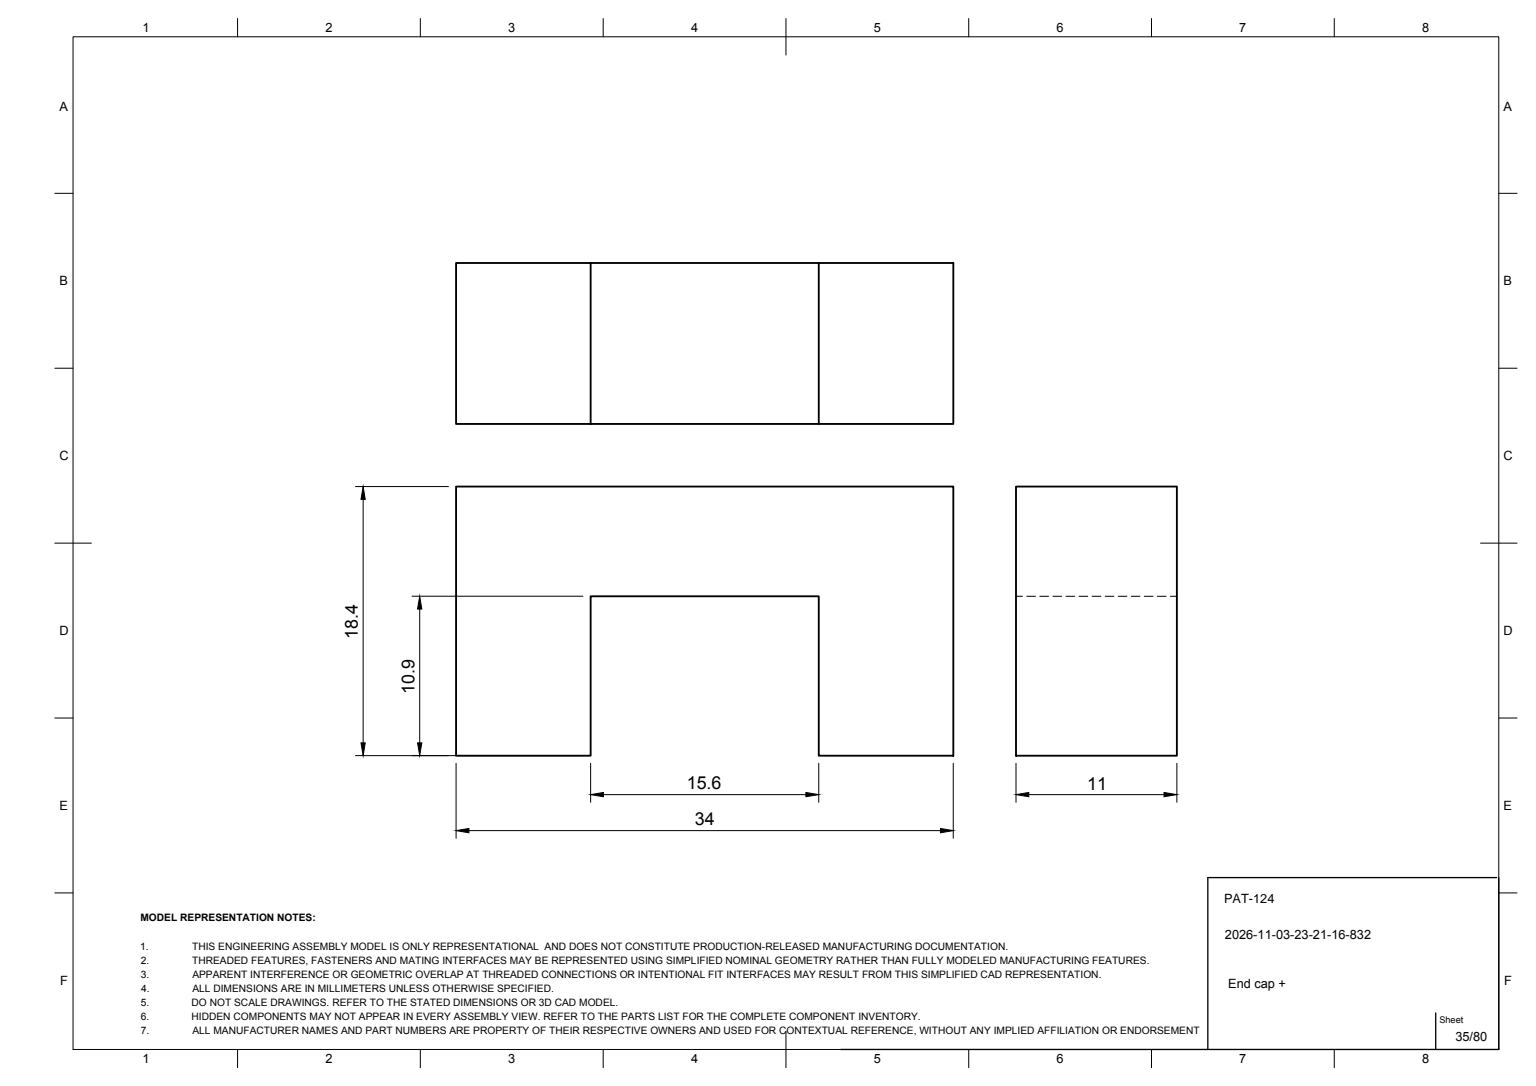
ISO-10303-21;
HEADER;
/* Generated by software containing ST-Developer
 * from STEP Tools, Inc. (www.steptools.com) 
 */

FILE_DESCRIPTION(
/* description */ ('XY cross-slide table'),
/* implementation_level */ '2;1');

FILE_NAME(
/* name */ 'End cap +.step',
/* time_stamp */ '2026-10-28T03:22:46-07:00',
/* author */ (''),
/* organization */ (''),
/* preprocessor_version */ 'ST-DEVELOPER v20.2',
/* originating_system */ 'Autodesk Translation Framework v15.17.0.0',
/* authorisation */ '');

FILE_SCHEMA (('AUTOMOTIVE_DESIGN { 1 0 10303 214 3 1 1 }'));
ENDSEC;

DATA;
#10=MECHANICAL_DESIGN_GEOMETRIC_PRESENTATION_REPRESENTATION('',(#1710),#62984);
#1529=SHAPE_REPRESENTATION_RELATIONSHIP('SRR','None',#63381,#1612);
#1612=ADVANCED_BREP_SHAPE_REPRESENTATION('',(#1823),#62918);
#1710=STYLED_ITEM('',(#63905),#1823);
#1823=MANIFOLD_SOLID_BREP('Body1',#23004);
#2457=PLANE('',#24689);
#2458=PLANE('',#24690);
#2459=PLANE('',#24691);
#2460=PLANE('',#24692);
#2461=PLANE('',#24693);
#2462=PLANE('',#24694);
#2463=PLANE('',#24695);
#2464=PLANE('',#24696);
#2465=PLANE('',#24697);
#2466=PLANE('',#24698);
#3186=FACE_OUTER_BOUND('',#4659,.T.);
#3187=FACE_OUTER_BOUND('',#4660,.T.);
#3188=FACE_OUTER_BOUND('',#4661,.T.);
#3189=FACE_OUTER_BOUND('',#4662,.T.);
#3190=FACE_OUTER_BOUND('',#4663,.T.);
#3191=FACE_OUTER_BOUND('',#4664,.T.);
#3192=FACE_OUTER_BOUND('',#4665,.T.);
#3193=FACE_OUTER_BOUND('',#4666,.T.);
#3194=FACE_OUTER_BOUND('',#4667,.T.);
#3195=FACE_OUTER_BOUND('',#4668,.T.);
#4659=EDGE_LOOP('',(#16324,#16325,#16326,#16327));
#4660=EDGE_LOOP('',(#16328,#16329,#16330,#16331));
#4661=EDGE_LOOP('',(#16332,#16333,#16334,#16335));
#4662=EDGE_LOOP('',(#16336,#16337,#16338,#16339));
#4663=EDGE_LOOP('',(#16340,#16341,#16342,#16343));
#4664=EDGE_LOOP('',(#16344,#16345,#16346,#16347));
#4665=EDGE_LOOP('',(#16348,#16349,#16350,#16351));
#4666=EDGE_LOOP('',(#16352,#16353,#16354,#16355));
#4667=EDGE_LOOP('',(#16356,#16357,#16358,#16359,#16360,#16361,#16362,#16363));
#4668=EDGE_LOOP('',(#16364,#16365,#16366,#16367,#16368,#16369,#16370,#16371));
#6255=LINE('',#35063,#7742);
#6256=LINE('',#35065,#7743);
#6257=LINE('',#35067,#7744);
#6258=LINE('',#35068,#7745);
#6259=LINE('',#35071,#7746);
#6260=LINE('',#35073,#7747);
#6261=LINE('',#35074,#7748);
#6262=LINE('',#35077,#7749);
#6263=LINE('',#35079,#7750);
#6264=LINE('',#35080,#7751);
#6265=LINE('',#35083,#7752);
#6266=LINE('',#35085,#7753);
#6267=LINE('',#35086,#7754);
#6268=LINE('',#35089,#7755);
#6269=LINE('',#35091,#7756);
#6270=LINE('',#35092,#7757);
#6271=LINE('',#35095,#7758);
#6272=LINE('',#35097,#7759);
#6273=LINE('',#35098,#7760);
#6274=LINE('',#35101,#7761);
#6275=LINE('',#35103,#7762);
#6276=LINE('',#35104,#7763);
#6277=LINE('',#35106,#7764);
#6278=LINE('',#35107,#7765);
#7742=VECTOR('',#28190,1.);
#7743=VECTOR('',#28191,1.);
#7744=VECTOR('',#28192,1.);
#7745=VECTOR('',#28193,1.);
#7746=VECTOR('',#28196,1.);
#7747=VECTOR('',#28197,1.);
#7748=VECTOR('',#28198,1.);
#7749=VECTOR('',#28201,1.);
#7750=VECTOR('',#28202,1.);
#7751=VECTOR('',#28203,1.);
#7752=VECTOR('',#28206,1.);
#7753=VECTOR('',#28207,1.);
#7754=VECTOR('',#28208,1.);
#7755=VECTOR('',#28211,1.);
#7756=VECTOR('',#28212,1.);
#7757=VECTOR('',#28213,1.);
#7758=VECTOR('',#28216,1.);
#7759=VECTOR('',#28217,1.);
#7760=VECTOR('',#28218,1.);
#7761=VECTOR('',#28221,1.);
#7762=VECTOR('',#28222,1.);
#7763=VECTOR('',#28223,1.);
#7764=VECTOR('',#28226,1.);
#7765=VECTOR('',#28227,1.);
#10261=VERTEX_POINT('',#35061);
#10262=VERTEX_POINT('',#35062);
#10263=VERTEX_POINT('',#35064);
#10264=VERTEX_POINT('',#35066);
#10265=VERTEX_POINT('',#35070);
#10266=VERTEX_POINT('',#35072);
#10267=VERTEX_POINT('',#35076);
#10268=VERTEX_POINT('',#35078);
#10269=VERTEX_POINT('',#35082);
#10270=VERTEX_POINT('',#35084);
#10271=VERTEX_POINT('',#35088);
#10272=VERTEX_POINT('',#35090);
#10273=VERTEX_POINT('',#35094);
#10274=VERTEX_POINT('',#35096);
#10275=VERTEX_POINT('',#35100);
#10276=VERTEX_POINT('',#35102);
#12546=EDGE_CURVE('',#10261,#10262,#6255,.T.);
#12547=EDGE_CURVE('',#10262,#10263,#6256,.T.);
#12548=EDGE_CURVE('',#10264,#10263,#6257,.T.);
#12549=EDGE_CURVE('',#10261,#10264,#6258,.T.);
#12550=EDGE_CURVE('',#10265,#10261,#6259,.T.);
#12551=EDGE_CURVE('',#10266,#10264,#6260,.T.);
#12552=EDGE_CURVE('',#10265,#10266,#6261,.T.);
#12553=EDGE_CURVE('',#10267,#10265,#6262,.T.);
#12554=EDGE_CURVE('',#10268,#10266,#6263,.T.);
#12555=EDGE_CURVE('',#10267,#10268,#6264,.T.);
#12556=EDGE_CURVE('',#10269,#10267,#6265,.T.);
#12557=EDGE_CURVE('',#10270,#10268,#6266,.T.);
#12558=EDGE_CURVE('',#10269,#10270,#6267,.T.);
#12559=EDGE_CURVE('',#10271,#10269,#6268,.T.);
#12560=EDGE_CURVE('',#10272,#10270,#6269,.T.);
#12561=EDGE_CURVE('',#10271,#10272,#6270,.T.);
#12562=EDGE_CURVE('',#10273,#10271,#6271,.T.);
#12563=EDGE_CURVE('',#10274,#10272,#6272,.T.);
#12564=EDGE_CURVE('',#10273,#10274,#6273,.T.);
#12565=EDGE_CURVE('',#10275,#10273,#6274,.T.);
#12566=EDGE_CURVE('',#10276,#10274,#6275,.T.);
#12567=EDGE_CURVE('',#10275,#10276,#6276,.T.);
#12568=EDGE_CURVE('',#10262,#10275,#6277,.T.);
#12569=EDGE_CURVE('',#10263,#10276,#6278,.T.);
#16324=ORIENTED_EDGE('',*,*,#12546,.T.);
#16325=ORIENTED_EDGE('',*,*,#12547,.T.);
#16326=ORIENTED_EDGE('',*,*,#12548,.F.);
#16327=ORIENTED_EDGE('',*,*,#12549,.F.);
#16328=ORIENTED_EDGE('',*,*,#12550,.T.);
#16329=ORIENTED_EDGE('',*,*,#12549,.T.);
#16330=ORIENTED_EDGE('',*,*,#12551,.F.);
#16331=ORIENTED_EDGE('',*,*,#12552,.F.);
#16332=ORIENTED_EDGE('',*,*,#12553,.T.);
#16333=ORIENTED_EDGE('',*,*,#12552,.T.);
#16334=ORIENTED_EDGE('',*,*,#12554,.F.);
#16335=ORIENTED_EDGE('',*,*,#12555,.F.);
#16336=ORIENTED_EDGE('',*,*,#12556,.T.);
#16337=ORIENTED_EDGE('',*,*,#12555,.T.);
#16338=ORIENTED_EDGE('',*,*,#12557,.F.);
#16339=ORIENTED_EDGE('',*,*,#12558,.F.);
#16340=ORIENTED_EDGE('',*,*,#12559,.T.);
#16341=ORIENTED_EDGE('',*,*,#12558,.T.);
#16342=ORIENTED_EDGE('',*,*,#12560,.F.);
#16343=ORIENTED_EDGE('',*,*,#12561,.F.);
#16344=ORIENTED_EDGE('',*,*,#12562,.T.);
#16345=ORIENTED_EDGE('',*,*,#12561,.T.);
#16346=ORIENTED_EDGE('',*,*,#12563,.F.);
#16347=ORIENTED_EDGE('',*,*,#12564,.F.);
#16348=ORIENTED_EDGE('',*,*,#12565,.T.);
#16349=ORIENTED_EDGE('',*,*,#12564,.T.);
#16350=ORIENTED_EDGE('',*,*,#12566,.F.);
#16351=ORIENTED_EDGE('',*,*,#12567,.F.);
#16352=ORIENTED_EDGE('',*,*,#12568,.T.);
#16353=ORIENTED_EDGE('',*,*,#12567,.T.);
#16354=ORIENTED_EDGE('',*,*,#12569,.F.);
#16355=ORIENTED_EDGE('',*,*,#12547,.F.);
#16356=ORIENTED_EDGE('',*,*,#12569,.T.);
#16357=ORIENTED_EDGE('',*,*,#12566,.T.);
#16358=ORIENTED_EDGE('',*,*,#12563,.T.);
#16359=ORIENTED_EDGE('',*,*,#12560,.T.);
#16360=ORIENTED_EDGE('',*,*,#12557,.T.);
#16361=ORIENTED_EDGE('',*,*,#12554,.T.);
#16362=ORIENTED_EDGE('',*,*,#12551,.T.);
#16363=ORIENTED_EDGE('',*,*,#12548,.T.);
#16364=ORIENTED_EDGE('',*,*,#12568,.F.);
#16365=ORIENTED_EDGE('',*,*,#12546,.F.);
#16366=ORIENTED_EDGE('',*,*,#12550,.F.);
#16367=ORIENTED_EDGE('',*,*,#12553,.F.);
#16368=ORIENTED_EDGE('',*,*,#12556,.F.);
#16369=ORIENTED_EDGE('',*,*,#12559,.F.);
#16370=ORIENTED_EDGE('',*,*,#12562,.F.);
#16371=ORIENTED_EDGE('',*,*,#12565,.F.);
#21967=ADVANCED_FACE('',(#3186),#2457,.T.);
#21968=ADVANCED_FACE('',(#3187),#2458,.T.);
#21969=ADVANCED_FACE('',(#3188),#2459,.T.);
#21970=ADVANCED_FACE('',(#3189),#2460,.T.);
#21971=ADVANCED_FACE('',(#3190),#2461,.T.);
#21972=ADVANCED_FACE('',(#3191),#2462,.T.);
#21973=ADVANCED_FACE('',(#3192),#2463,.T.);
#21974=ADVANCED_FACE('',(#3193),#2464,.T.);
#21975=ADVANCED_FACE('',(#3194),#2465,.T.);
#21976=ADVANCED_FACE('',(#3195),#2466,.F.);
#23004=CLOSED_SHELL('',(#21967,#21968,#21969,#21970,#21971,#21972,#21973,
#21974,#21975,#21976));
#24688=AXIS2_PLACEMENT_3D('',#35059,#28186,#28187);
#24689=AXIS2_PLACEMENT_3D('',#35060,#28188,#28189);
#24690=AXIS2_PLACEMENT_3D('',#35069,#28194,#28195);
#24691=AXIS2_PLACEMENT_3D('',#35075,#28199,#28200);
#24692=AXIS2_PLACEMENT_3D('',#35081,#28204,#28205);
#24693=AXIS2_PLACEMENT_3D('',#35087,#28209,#28210);
#24694=AXIS2_PLACEMENT_3D('',#35093,#28214,#28215);
#24695=AXIS2_PLACEMENT_3D('',#35099,#28219,#28220);
#24696=AXIS2_PLACEMENT_3D('',#35105,#28224,#28225);
#24697=AXIS2_PLACEMENT_3D('',#35108,#28228,#28229);
#24698=AXIS2_PLACEMENT_3D('',#35109,#28230,#28231);
#28186=DIRECTION('axis',(0.,0.,1.));
#28187=DIRECTION('refdir',(1.,0.,0.));
#28188=DIRECTION('center_axis',(0.,0.,1.));
#28189=DIRECTION('ref_axis',(0.,-1.,0.));
#28190=DIRECTION('',(0.,-1.,0.));
#28191=DIRECTION('',(1.,0.,0.));
#28192=DIRECTION('',(0.,-1.,0.));
#28193=DIRECTION('',(1.,0.,0.));
#28194=DIRECTION('center_axis',(0.,1.,0.));
#28195=DIRECTION('ref_axis',(0.,0.,1.));
#28196=DIRECTION('',(0.,0.,1.));
#28197=DIRECTION('',(0.,0.,1.));
#28198=DIRECTION('',(1.,0.,0.));
#28199=DIRECTION('center_axis',(0.,0.,-1.));
#28200=DIRECTION('ref_axis',(0.,1.,0.));
#28201=DIRECTION('',(0.,1.,0.));
#28202=DIRECTION('',(0.,1.,0.));
#28203=DIRECTION('',(1.,0.,0.));
#28204=DIRECTION('center_axis',(0.,-1.,0.));
#28205=DIRECTION('ref_axis',(0.,0.,-1.));
#28206=DIRECTION('',(0.,0.,-1.));
#28207=DIRECTION('',(0.,0.,-1.));
#28208=DIRECTION('',(1.,0.,0.));
#28209=DIRECTION('center_axis',(0.,0.,-1.));
#28210=DIRECTION('ref_axis',(0.,1.,0.));
#28211=DIRECTION('',(0.,1.,0.));
#28212=DIRECTION('',(0.,1.,0.));
#28213=DIRECTION('',(1.,0.,0.));
#28214=DIRECTION('center_axis',(0.,1.,0.));
#28215=DIRECTION('ref_axis',(0.,0.,1.));
#28216=DIRECTION('',(0.,0.,1.));
#28217=DIRECTION('',(0.,0.,1.));
#28218=DIRECTION('',(1.,0.,0.));
#28219=DIRECTION('center_axis',(0.,0.,-1.));
#28220=DIRECTION('ref_axis',(0.,1.,0.));
#28221=DIRECTION('',(0.,1.,0.));
#28222=DIRECTION('',(0.,1.,0.));
#28223=DIRECTION('',(1.,0.,0.));
#28224=DIRECTION('center_axis',(0.,-1.,0.));
#28225=DIRECTION('ref_axis',(0.,0.,-1.));
#28226=DIRECTION('',(0.,0.,-1.));
#28227=DIRECTION('',(0.,0.,-1.));
#28228=DIRECTION('center_axis',(1.,0.,0.));
#28229=DIRECTION('ref_axis',(0.,0.,-1.));
#28230=DIRECTION('center_axis',(1.,0.,0.));
#28231=DIRECTION('ref_axis',(0.,0.,-1.));
#35059=CARTESIAN_POINT('',(0.,0.,0.));
#35060=CARTESIAN_POINT('Origin',(1.97,1.7,2.3));
#35061=CARTESIAN_POINT('',(1.97,1.7,2.3));
#35062=CARTESIAN_POINT('',(1.97,-1.7,2.3));
#35063=CARTESIAN_POINT('',(1.97,1.7,2.3));
#35064=CARTESIAN_POINT('',(3.07,-1.7,2.3));
#35065=CARTESIAN_POINT('',(1.97,-1.7,2.3));
#35066=CARTESIAN_POINT('',(3.07,1.7,2.3));
#35067=CARTESIAN_POINT('',(3.07,1.7,2.3));
#35068=CARTESIAN_POINT('',(1.97,1.7,2.3));
#35069=CARTESIAN_POINT('Origin',(1.97,1.7,0.46));
#35070=CARTESIAN_POINT('',(1.97,1.7,0.46));
#35071=CARTESIAN_POINT('',(1.97,1.7,0.46));
#35072=CARTESIAN_POINT('',(3.07,1.7,0.46));
#35073=CARTESIAN_POINT('',(3.07,1.7,0.46));
#35074=CARTESIAN_POINT('',(1.97,1.7,0.46));
#35075=CARTESIAN_POINT('Origin',(1.97,0.78,0.46));
#35076=CARTESIAN_POINT('',(1.97,0.78,0.46));
#35077=CARTESIAN_POINT('',(1.97,0.78,0.46));
#35078=CARTESIAN_POINT('',(3.07,0.78,0.46));
#35079=CARTESIAN_POINT('',(3.07,0.78,0.46));
#35080=CARTESIAN_POINT('',(1.97,0.78,0.46));
#35081=CARTESIAN_POINT('Origin',(1.97,0.78,1.55));
#35082=CARTESIAN_POINT('',(1.97,0.78,1.55));
#35083=CARTESIAN_POINT('',(1.97,0.78,1.55));
#35084=CARTESIAN_POINT('',(3.07,0.78,1.55));
#35085=CARTESIAN_POINT('',(3.07,0.78,1.55));
#35086=CARTESIAN_POINT('',(1.97,0.78,1.55));
#35087=CARTESIAN_POINT('Origin',(1.97,-0.78,1.55));
#35088=CARTESIAN_POINT('',(1.97,-0.78,1.55));
#35089=CARTESIAN_POINT('',(1.97,-0.78,1.55));
#35090=CARTESIAN_POINT('',(3.07,-0.78,1.55));
#35091=CARTESIAN_POINT('',(3.07,-0.78,1.55));
#35092=CARTESIAN_POINT('',(1.97,-0.78,1.55));
#35093=CARTESIAN_POINT('Origin',(1.97,-0.78,0.46));
#35094=CARTESIAN_POINT('',(1.97,-0.78,0.46));
#35095=CARTESIAN_POINT('',(1.97,-0.78,0.46));
#35096=CARTESIAN_POINT('',(3.07,-0.78,0.46));
#35097=CARTESIAN_POINT('',(3.07,-0.78,0.46));
#35098=CARTESIAN_POINT('',(1.97,-0.78,0.46));
#35099=CARTESIAN_POINT('Origin',(1.97,-1.7,0.46));
#35100=CARTESIAN_POINT('',(1.97,-1.7,0.46));
#35101=CARTESIAN_POINT('',(1.97,-1.7,0.46));
#35102=CARTESIAN_POINT('',(3.07,-1.7,0.46));
#35103=CARTESIAN_POINT('',(3.07,-1.7,0.46));
#35104=CARTESIAN_POINT('',(1.97,-1.7,0.46));
#35105=CARTESIAN_POINT('Origin',(1.97,-1.7,2.3));
#35106=CARTESIAN_POINT('',(1.97,-1.7,2.3));
#35107=CARTESIAN_POINT('',(3.07,-1.7,2.3));
#35108=CARTESIAN_POINT('Origin',(3.07,0.,1.38));
#35109=CARTESIAN_POINT('Origin',(1.97,0.,1.38));
#62819=UNCERTAINTY_MEASURE_WITH_UNIT(LENGTH_MEASURE(0.001),#62985,
'DISTANCE_ACCURACY_VALUE',
'Maximum model space distance between geometric entities at asserted c
onnectivities');
#62885=UNCERTAINTY_MEASURE_WITH_UNIT(LENGTH_MEASURE(0.001),#62985,
'DISTANCE_ACCURACY_VALUE',
'Maximum model space distance between geometric entities at asserted c
onnectivities');
#62918=(
GEOMETRIC_REPRESENTATION_CONTEXT(3)
GLOBAL_UNCERTAINTY_ASSIGNED_CONTEXT((#62819))
GLOBAL_UNIT_ASSIGNED_CONTEXT((#62985,#62987,#62988))
REPRESENTATION_CONTEXT('','3D')
);
#62984=(
GEOMETRIC_REPRESENTATION_CONTEXT(3)
GLOBAL_UNCERTAINTY_ASSIGNED_CONTEXT((#62885))
GLOBAL_UNIT_ASSIGNED_CONTEXT((#62985,#62987,#62988))
REPRESENTATION_CONTEXT('','3D')
);
#62985=(
LENGTH_UNIT()
NAMED_UNIT(*)
SI_UNIT(.CENTI.,.METRE.)
);
#62987=(
NAMED_UNIT(*)
PLANE_ANGLE_UNIT()
SI_UNIT($,.RADIAN.)
);
#62988=(
NAMED_UNIT(*)
SI_UNIT($,.STERADIAN.)
SOLID_ANGLE_UNIT()
);
#63021=SHAPE_DEFINITION_REPRESENTATION(#63129,#63381);
#63129=PRODUCT_DEFINITION_SHAPE('',$,#63480);
#63381=SHAPE_REPRESENTATION('',(#24688),#62918);
#63447=PRODUCT_DEFINITION_CONTEXT('part definition',#63743,'design');
#63480=PRODUCT_DEFINITION('End cap +','End cap +',#63578,#63447);
#63578=PRODUCT_DEFINITION_FORMATION('',$,#63777);
#63743=APPLICATION_CONTEXT(
'Core Data for Automotive Mechanical Design Process');
#63744=PRODUCT_CONTEXT('part definition',#63743,'mechanical');
#63777=PRODUCT('End cap +','End cap +','End cap +',(#63744));
#63899=COLOUR_RGB('Sky Blue',0.24,0.69,0.87);
#63900=FILL_AREA_STYLE_COLOUR('',#63899);
#63901=FILL_AREA_STYLE('',(#63900));
#63902=SURFACE_STYLE_FILL_AREA(#63901);
#63903=SURFACE_SIDE_STYLE('',(#63902));
#63904=SURFACE_STYLE_USAGE(.BOTH.,#63903);
#63905=PRESENTATION_STYLE_ASSIGNMENT((#63904));
ENDSEC;
END-ISO-10303-21;
